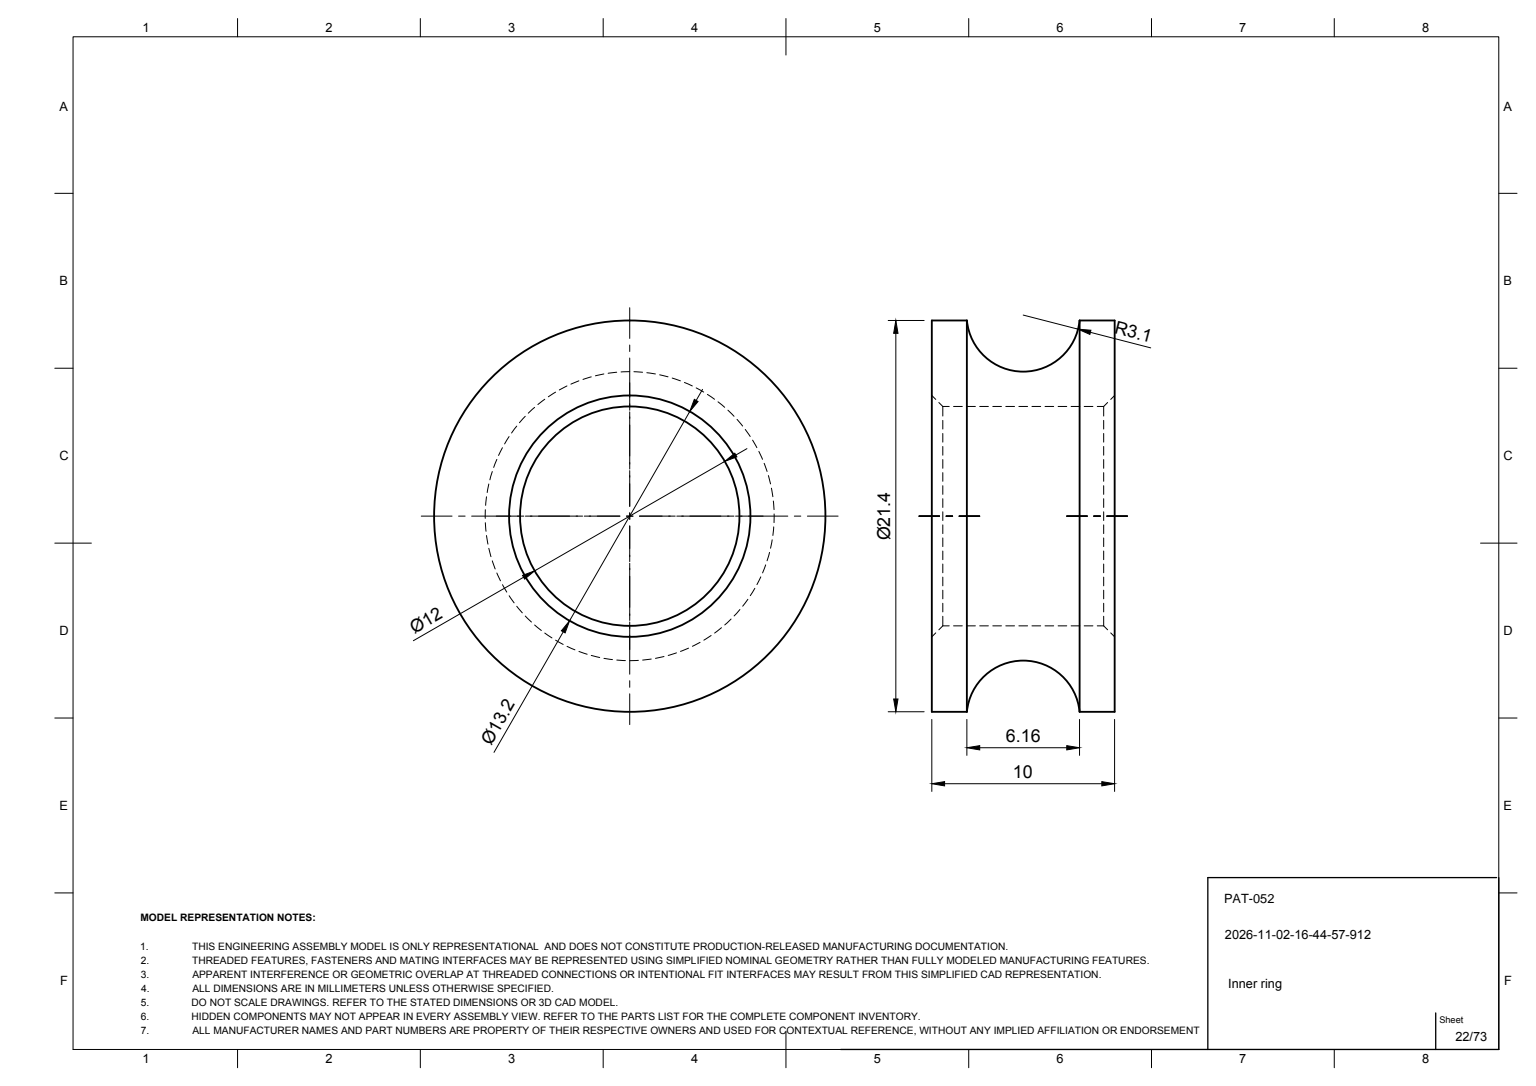
ISO-10303-21;
HEADER;
/* Generated by software containing ST-Developer
 * from STEP Tools, Inc. (www.steptools.com) 
 */

FILE_DESCRIPTION(
/* description */ ('Hand-crank gear train demonstrator'),
/* implementation_level */ '2;1');

FILE_NAME(
/* name */ 'Inner ring.step',
/* time_stamp */ '2026-10-28T03:22:13-07:00',
/* author */ (''),
/* organization */ (''),
/* preprocessor_version */ 'ST-DEVELOPER v20.2',
/* originating_system */ 'Autodesk Translation Framework v15.17.0.0',
/* authorisation */ '');

FILE_SCHEMA (('AUTOMOTIVE_DESIGN { 1 0 10303 214 3 1 1 }'));
ENDSEC;

DATA;
#10=MECHANICAL_DESIGN_GEOMETRIC_PRESENTATION_REPRESENTATION('',(#1200),#62758);
#1021=TOROIDAL_SURFACE('',#17486,1.1,0.309556);
#1028=CONICAL_SURFACE('',#17497,0.63,0.785398163397448);
#1029=CONICAL_SURFACE('',#17504,0.63,0.785398163397448);
#1072=SHAPE_REPRESENTATION_RELATIONSHIP('SRR','None',#63045,#1136);
#1136=ADVANCED_BREP_SHAPE_REPRESENTATION('',(#1278),#62699);
#1200=STYLED_ITEM('',(#63462),#1278);
#1278=MANIFOLD_SOLID_BREP('Body1',#16381);
#1487=FACE_BOUND('',#3347,.T.);
#1488=FACE_BOUND('',#3350,.T.);
#1682=PLANE('',#17499);
#1683=PLANE('',#17502);
#2261=FACE_OUTER_BOUND('',#3342,.T.);
#2262=FACE_OUTER_BOUND('',#3343,.T.);
#2263=FACE_OUTER_BOUND('',#3344,.T.);
#2264=FACE_OUTER_BOUND('',#3345,.T.);
#2265=FACE_OUTER_BOUND('',#3346,.T.);
#2266=FACE_OUTER_BOUND('',#3348,.T.);
#2267=FACE_OUTER_BOUND('',#3349,.T.);
#2268=FACE_OUTER_BOUND('',#3351,.T.);
#3342=EDGE_LOOP('',(#11459,#11460,#11461,#11462,#11463,#11464));
#3343=EDGE_LOOP('',(#11465,#11466,#11467,#11468,#11469));
#3344=EDGE_LOOP('',(#11470,#11471,#11472,#11473));
#3345=EDGE_LOOP('',(#11474,#11475,#11476,#11477));
#3346=EDGE_LOOP('',(#11478));
#3347=EDGE_LOOP('',(#11479));
#3348=EDGE_LOOP('',(#11480,#11481,#11482,#11483,#11484));
#3349=EDGE_LOOP('',(#11485));
#3350=EDGE_LOOP('',(#11486));
#3351=EDGE_LOOP('',(#11487,#11488,#11489,#11490));
#4423=LINE('',#23993,#5555);
#4424=LINE('',#23999,#5556);
#4425=LINE('',#24003,#5557);
#4426=LINE('',#24009,#5558);
#4427=LINE('',#24014,#5559);
#5555=VECTOR('',#19638,1.070235);
#5556=VECTOR('',#19645,0.6);
#5557=VECTOR('',#19650,0.63);
#5558=VECTOR('',#19659,1.070235);
#5559=VECTOR('',#19666,0.63);
#6725=CIRCLE('',#17487,1.070235);
#6726=CIRCLE('',#17488,1.070235);
#6727=CIRCLE('',#17489,0.309556);
#6728=CIRCLE('',#17490,1.070235);
#6729=CIRCLE('',#17491,1.070235);
#6730=CIRCLE('',#17493,1.070235);
#6731=CIRCLE('',#17495,0.6);
#6732=CIRCLE('',#17496,0.6);
#6733=CIRCLE('',#17498,0.66);
#6734=CIRCLE('',#17501,1.070235);
#6735=CIRCLE('',#17503,0.66);
#7419=VERTEX_POINT('',#23982);
#7420=VERTEX_POINT('',#23983);
#7421=VERTEX_POINT('',#23986);
#7422=VERTEX_POINT('',#23988);
#7423=VERTEX_POINT('',#23992);
#7424=VERTEX_POINT('',#23996);
#7425=VERTEX_POINT('',#23998);
#7426=VERTEX_POINT('',#24002);
#7427=VERTEX_POINT('',#24007);
#7428=VERTEX_POINT('',#24011);
#8981=EDGE_CURVE('',#7419,#7420,#6725,.T.);
#8982=EDGE_CURVE('',#7420,#7419,#6726,.T.);
#8983=EDGE_CURVE('',#7420,#7421,#6727,.T.);
#8984=EDGE_CURVE('',#7422,#7421,#6728,.T.);
#8985=EDGE_CURVE('',#7421,#7422,#6729,.T.);
#8986=EDGE_CURVE('',#7422,#7423,#4423,.T.);
#8987=EDGE_CURVE('',#7423,#7423,#6730,.T.);
#8988=EDGE_CURVE('',#7424,#7424,#6731,.T.);
#8989=EDGE_CURVE('',#7424,#7425,#4424,.T.);
#8990=EDGE_CURVE('',#7425,#7425,#6732,.T.);
#8991=EDGE_CURVE('',#7425,#7426,#4425,.T.);
#8992=EDGE_CURVE('',#7426,#7426,#6733,.T.);
#8993=EDGE_CURVE('',#7427,#7427,#6734,.T.);
#8994=EDGE_CURVE('',#7427,#7419,#4426,.T.);
#8995=EDGE_CURVE('',#7428,#7428,#6735,.T.);
#8996=EDGE_CURVE('',#7428,#7424,#4427,.T.);
#11459=ORIENTED_EDGE('',*,*,#8981,.F.);
#11460=ORIENTED_EDGE('',*,*,#8982,.F.);
#11461=ORIENTED_EDGE('',*,*,#8983,.T.);
#11462=ORIENTED_EDGE('',*,*,#8984,.F.);
#11463=ORIENTED_EDGE('',*,*,#8985,.F.);
#11464=ORIENTED_EDGE('',*,*,#8983,.F.);
#11465=ORIENTED_EDGE('',*,*,#8984,.T.);
#11466=ORIENTED_EDGE('',*,*,#8985,.T.);
#11467=ORIENTED_EDGE('',*,*,#8986,.T.);
#11468=ORIENTED_EDGE('',*,*,#8987,.T.);
#11469=ORIENTED_EDGE('',*,*,#8986,.F.);
#11470=ORIENTED_EDGE('',*,*,#8988,.T.);
#11471=ORIENTED_EDGE('',*,*,#8989,.T.);
#11472=ORIENTED_EDGE('',*,*,#8990,.F.);
#11473=ORIENTED_EDGE('',*,*,#8989,.F.);
#11474=ORIENTED_EDGE('',*,*,#8990,.T.);
#11475=ORIENTED_EDGE('',*,*,#8991,.T.);
#11476=ORIENTED_EDGE('',*,*,#8992,.F.);
#11477=ORIENTED_EDGE('',*,*,#8991,.F.);
#11478=ORIENTED_EDGE('',*,*,#8987,.F.);
#11479=ORIENTED_EDGE('',*,*,#8992,.T.);
#11480=ORIENTED_EDGE('',*,*,#8993,.F.);
#11481=ORIENTED_EDGE('',*,*,#8994,.T.);
#11482=ORIENTED_EDGE('',*,*,#8981,.T.);
#11483=ORIENTED_EDGE('',*,*,#8982,.T.);
#11484=ORIENTED_EDGE('',*,*,#8994,.F.);
#11485=ORIENTED_EDGE('',*,*,#8993,.T.);
#11486=ORIENTED_EDGE('',*,*,#8995,.F.);
#11487=ORIENTED_EDGE('',*,*,#8995,.T.);
#11488=ORIENTED_EDGE('',*,*,#8996,.T.);
#11489=ORIENTED_EDGE('',*,*,#8988,.F.);
#11490=ORIENTED_EDGE('',*,*,#8996,.F.);
#15253=CYLINDRICAL_SURFACE('',#17492,1.070235);
#15254=CYLINDRICAL_SURFACE('',#17494,0.6);
#15255=CYLINDRICAL_SURFACE('',#17500,1.070235);
#15571=ADVANCED_FACE('',(#2261),#1021,.F.);
#15572=ADVANCED_FACE('',(#2262),#15253,.T.);
#15573=ADVANCED_FACE('',(#2263),#15254,.F.);
#15574=ADVANCED_FACE('',(#2264),#1028,.F.);
#15575=ADVANCED_FACE('',(#2265,#1487),#1682,.T.);
#15576=ADVANCED_FACE('',(#2266),#15255,.T.);
#15577=ADVANCED_FACE('',(#2267,#1488),#1683,.T.);
#15578=ADVANCED_FACE('',(#2268),#1029,.F.);
#16381=CLOSED_SHELL('',(#15571,#15572,#15573,#15574,#15575,#15576,#15577,
#15578));
#17485=AXIS2_PLACEMENT_3D('',#23980,#19622,#19623);
#17486=AXIS2_PLACEMENT_3D('',#23981,#19624,#19625);
#17487=AXIS2_PLACEMENT_3D('',#23984,#19626,#19627);
#17488=AXIS2_PLACEMENT_3D('',#23985,#19628,#19629);
#17489=AXIS2_PLACEMENT_3D('',#23987,#19630,#19631);
#17490=AXIS2_PLACEMENT_3D('',#23989,#19632,#19633);
#17491=AXIS2_PLACEMENT_3D('',#23990,#19634,#19635);
#17492=AXIS2_PLACEMENT_3D('',#23991,#19636,#19637);
#17493=AXIS2_PLACEMENT_3D('',#23994,#19639,#19640);
#17494=AXIS2_PLACEMENT_3D('',#23995,#19641,#19642);
#17495=AXIS2_PLACEMENT_3D('',#23997,#19643,#19644);
#17496=AXIS2_PLACEMENT_3D('',#24000,#19646,#19647);
#17497=AXIS2_PLACEMENT_3D('',#24001,#19648,#19649);
#17498=AXIS2_PLACEMENT_3D('',#24004,#19651,#19652);
#17499=AXIS2_PLACEMENT_3D('',#24005,#19653,#19654);
#17500=AXIS2_PLACEMENT_3D('',#24006,#19655,#19656);
#17501=AXIS2_PLACEMENT_3D('',#24008,#19657,#19658);
#17502=AXIS2_PLACEMENT_3D('',#24010,#19660,#19661);
#17503=AXIS2_PLACEMENT_3D('',#24012,#19662,#19663);
#17504=AXIS2_PLACEMENT_3D('',#24013,#19664,#19665);
#19622=DIRECTION('axis',(0.,0.,1.));
#19623=DIRECTION('refdir',(1.,0.,0.));
#19624=DIRECTION('center_axis',(0.,-1.,0.));
#19625=DIRECTION('ref_axis',(0.,0.,-1.));
#19626=DIRECTION('center_axis',(0.,-1.,0.));
#19627=DIRECTION('ref_axis',(1.,0.,0.));
#19628=DIRECTION('center_axis',(0.,-1.,0.));
#19629=DIRECTION('ref_axis',(1.,0.,0.));
#19630=DIRECTION('center_axis',(1.,0.,1.22464679914735E-16));
#19631=DIRECTION('ref_axis',(-1.22464679914735E-16,0.,1.));
#19632=DIRECTION('center_axis',(0.,1.,0.));
#19633=DIRECTION('ref_axis',(1.,0.,0.));
#19634=DIRECTION('center_axis',(0.,1.,0.));
#19635=DIRECTION('ref_axis',(1.,0.,0.));
#19636=DIRECTION('center_axis',(0.,-1.,0.));
#19637=DIRECTION('ref_axis',(1.,0.,0.));
#19638=DIRECTION('',(0.,1.,0.));
#19639=DIRECTION('center_axis',(0.,-1.,0.));
#19640=DIRECTION('ref_axis',(1.,0.,0.));
#19641=DIRECTION('center_axis',(0.,-1.,0.));
#19642=DIRECTION('ref_axis',(1.,0.,0.));
#19643=DIRECTION('center_axis',(0.,-1.,0.));
#19644=DIRECTION('ref_axis',(1.,0.,0.));
#19645=DIRECTION('',(0.,1.,0.));
#19646=DIRECTION('center_axis',(0.,-1.,0.));
#19647=DIRECTION('ref_axis',(1.,0.,0.));
#19648=DIRECTION('center_axis',(0.,1.,0.));
#19649=DIRECTION('ref_axis',(1.,0.,0.));
#19650=DIRECTION('',(-0.707106781186548,0.707106781186547,-8.65956056235493E-17));
#19651=DIRECTION('center_axis',(0.,-1.,0.));
#19652=DIRECTION('ref_axis',(1.,0.,0.));
#19653=DIRECTION('center_axis',(0.,1.,0.));
#19654=DIRECTION('ref_axis',(0.,0.,1.));
#19655=DIRECTION('center_axis',(0.,-1.,0.));
#19656=DIRECTION('ref_axis',(1.,0.,0.));
#19657=DIRECTION('center_axis',(0.,-1.,0.));
#19658=DIRECTION('ref_axis',(1.,0.,0.));
#19659=DIRECTION('',(0.,1.,0.));
#19660=DIRECTION('center_axis',(0.,-1.,0.));
#19661=DIRECTION('ref_axis',(0.,0.,-1.));
#19662=DIRECTION('center_axis',(0.,-1.,0.));
#19663=DIRECTION('ref_axis',(1.,0.,0.));
#19664=DIRECTION('center_axis',(0.,-1.,0.));
#19665=DIRECTION('ref_axis',(1.,0.,0.));
#19666=DIRECTION('',(0.707106781186548,0.707106781186547,8.65956056235493E-17));
#23980=CARTESIAN_POINT('',(0.,0.,0.));
#23981=CARTESIAN_POINT('Origin',(0.,0.,0.));
#23982=CARTESIAN_POINT('',(-1.070235,-0.308121667383195,-1.31065986708547E-16));
#23983=CARTESIAN_POINT('',(-1.31065986708547E-16,-0.308121667383195,1.070235));
#23984=CARTESIAN_POINT('Origin',(0.,-0.308121667383195,0.));
#23985=CARTESIAN_POINT('Origin',(0.,-0.308121667383195,0.));
#23986=CARTESIAN_POINT('',(-1.31065986708547E-16,0.308121667383195,1.070235));
#23987=CARTESIAN_POINT('Origin',(-1.34711147906209E-16,0.,1.1));
#23988=CARTESIAN_POINT('',(-1.070235,0.308121667383195,1.31065986708547E-16));
#23989=CARTESIAN_POINT('Origin',(0.,0.308121667383195,0.));
#23990=CARTESIAN_POINT('Origin',(0.,0.308121667383195,0.));
#23991=CARTESIAN_POINT('Origin',(0.,0.,0.));
#23992=CARTESIAN_POINT('',(-1.070235,0.5,-1.31065986708547E-16));
#23993=CARTESIAN_POINT('',(-1.070235,0.,-1.31065986708547E-16));
#23994=CARTESIAN_POINT('Origin',(0.,0.5,0.));
#23995=CARTESIAN_POINT('Origin',(0.,0.,0.));
#23996=CARTESIAN_POINT('',(-0.6,-0.44,-7.34788079488412E-17));
#23997=CARTESIAN_POINT('Origin',(0.,-0.44,0.));
#23998=CARTESIAN_POINT('',(-0.6,0.44,-7.34788079488412E-17));
#23999=CARTESIAN_POINT('',(-0.6,0.,-7.34788079488412E-17));
#24000=CARTESIAN_POINT('Origin',(0.,0.44,0.));
#24001=CARTESIAN_POINT('Origin',(0.,0.47,0.));
#24002=CARTESIAN_POINT('',(-0.66,0.5,-8.08266887437253E-17));
#24003=CARTESIAN_POINT('',(-0.63,0.47,-7.71527483462832E-17));
#24004=CARTESIAN_POINT('Origin',(0.,0.5,0.));
#24005=CARTESIAN_POINT('Origin',(1.070235,0.5,0.));
#24006=CARTESIAN_POINT('Origin',(0.,0.,0.));
#24007=CARTESIAN_POINT('',(-1.070235,-0.5,-1.31065986708547E-16));
#24008=CARTESIAN_POINT('Origin',(0.,-0.5,0.));
#24009=CARTESIAN_POINT('',(-1.070235,0.,-1.31065986708547E-16));
#24010=CARTESIAN_POINT('Origin',(0.66,-0.5,0.));
#24011=CARTESIAN_POINT('',(-0.66,-0.5,-8.08266887437253E-17));
#24012=CARTESIAN_POINT('Origin',(0.,-0.5,0.));
#24013=CARTESIAN_POINT('Origin',(0.,-0.47,0.));
#24014=CARTESIAN_POINT('',(-0.63,-0.47,-7.71527483462832E-17));
#62625=UNCERTAINTY_MEASURE_WITH_UNIT(LENGTH_MEASURE(0.001),#62759,
'DISTANCE_ACCURACY_VALUE',
'Maximum model space distance between geometric entities at asserted c
onnectivities');
#62684=UNCERTAINTY_MEASURE_WITH_UNIT(LENGTH_MEASURE(0.001),#62759,
'DISTANCE_ACCURACY_VALUE',
'Maximum model space distance between geometric entities at asserted c
onnectivities');
#62699=(
GEOMETRIC_REPRESENTATION_CONTEXT(3)
GLOBAL_UNCERTAINTY_ASSIGNED_CONTEXT((#62625))
GLOBAL_UNIT_ASSIGNED_CONTEXT((#62759,#62761,#62762))
REPRESENTATION_CONTEXT('','3D')
);
#62758=(
GEOMETRIC_REPRESENTATION_CONTEXT(3)
GLOBAL_UNCERTAINTY_ASSIGNED_CONTEXT((#62684))
GLOBAL_UNIT_ASSIGNED_CONTEXT((#62759,#62761,#62762))
REPRESENTATION_CONTEXT('','3D')
);
#62759=(
LENGTH_UNIT()
NAMED_UNIT(*)
SI_UNIT(.CENTI.,.METRE.)
);
#62761=(
NAMED_UNIT(*)
PLANE_ANGLE_UNIT()
SI_UNIT($,.RADIAN.)
);
#62762=(
NAMED_UNIT(*)
SI_UNIT($,.STERADIAN.)
SOLID_ANGLE_UNIT()
);
#62777=SHAPE_DEFINITION_REPRESENTATION(#62850,#63045);
#62850=PRODUCT_DEFINITION_SHAPE('',$,#63119);
#63045=SHAPE_REPRESENTATION('',(#17485),#62699);
#63104=PRODUCT_DEFINITION_CONTEXT('part definition',#63325,'design');
#63119=PRODUCT_DEFINITION('Inner ring','Inner ring',#63192,#63104);
#63192=PRODUCT_DEFINITION_FORMATION('',$,#63341);
#63325=APPLICATION_CONTEXT(
'Core Data for Automotive Mechanical Design Process');
#63326=PRODUCT_CONTEXT('part definition',#63325,'mechanical');
#63341=PRODUCT('Inner ring','Inner ring','Inner ring',(#63326));
#63456=COLOUR_RGB('Grey',0.48,0.52,0.57);
#63457=FILL_AREA_STYLE_COLOUR('',#63456);
#63458=FILL_AREA_STYLE('',(#63457));
#63459=SURFACE_STYLE_FILL_AREA(#63458);
#63460=SURFACE_SIDE_STYLE('',(#63459));
#63461=SURFACE_STYLE_USAGE(.BOTH.,#63460);
#63462=PRESENTATION_STYLE_ASSIGNMENT((#63461));
ENDSEC;
END-ISO-10303-21;
